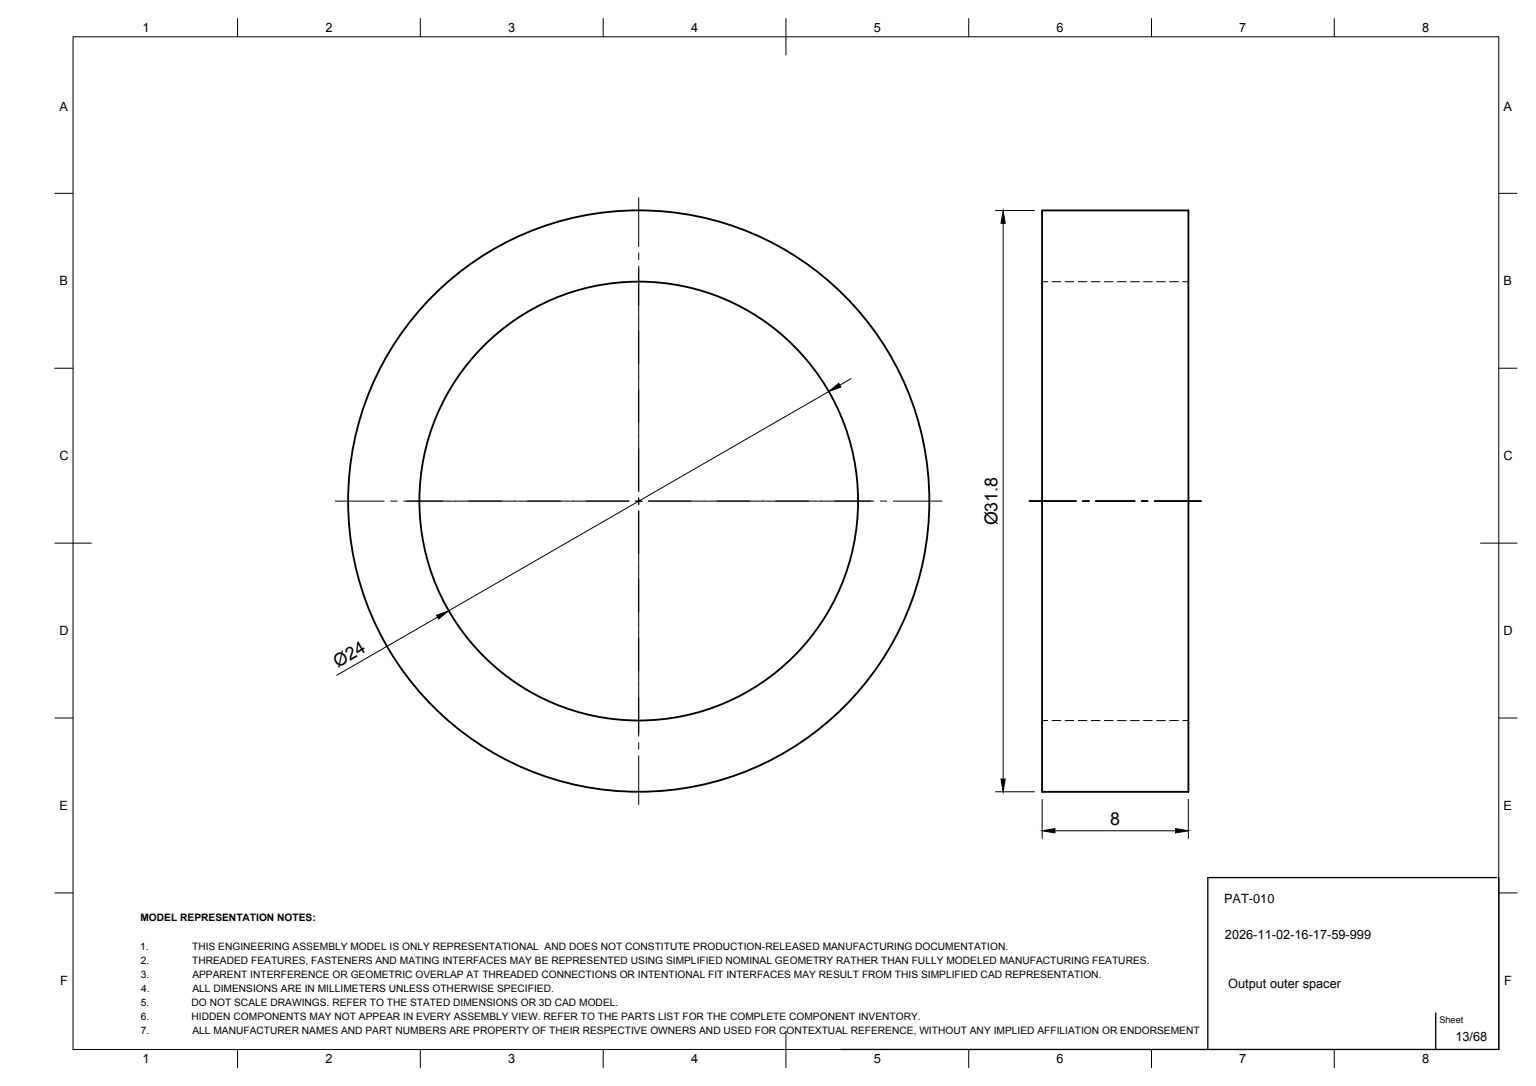
ISO-10303-21;
HEADER;
/* Generated by software containing ST-Developer
 * from STEP Tools, Inc. (www.steptools.com) 
 */

FILE_DESCRIPTION(
/* description */ ('Belt conveyor head drive unit'),
/* implementation_level */ '2;1');

FILE_NAME(
/* name */ 'Output outer spacer.step',
/* time_stamp */ '2026-10-28T03:26:19-07:00',
/* author */ (''),
/* organization */ (''),
/* preprocessor_version */ 'ST-DEVELOPER v20.2',
/* originating_system */ 'Autodesk Translation Framework v15.17.0.0',
/* authorisation */ '');

FILE_SCHEMA (('AUTOMOTIVE_DESIGN { 1 0 10303 214 3 1 1 }'));
ENDSEC;

DATA;
#10=MECHANICAL_DESIGN_GEOMETRIC_PRESENTATION_REPRESENTATION('',(#859),#27069);
#721=SHAPE_REPRESENTATION_RELATIONSHIP('SRR','None',#27365,#790);
#790=ADVANCED_BREP_SHAPE_REPRESENTATION('',(#944),#27007);
#859=STYLED_ITEM('',(#27811),#944);
#944=MANIFOLD_SOLID_BREP('Body1',#13724);
#1084=FACE_BOUND('',#2660,.T.);
#1085=FACE_BOUND('',#2662,.T.);
#1356=PLANE('',#14885);
#1357=PLANE('',#14886);
#1785=FACE_OUTER_BOUND('',#2657,.T.);
#1786=FACE_OUTER_BOUND('',#2658,.T.);
#1787=FACE_OUTER_BOUND('',#2659,.T.);
#1788=FACE_OUTER_BOUND('',#2661,.T.);
#2657=EDGE_LOOP('',(#9642,#9643,#9644,#9645));
#2658=EDGE_LOOP('',(#9646,#9647,#9648,#9649));
#2659=EDGE_LOOP('',(#9650));
#2660=EDGE_LOOP('',(#9651));
#2661=EDGE_LOOP('',(#9652));
#2662=EDGE_LOOP('',(#9653));
#3690=LINE('',#21711,#4482);
#3691=LINE('',#21717,#4483);
#4482=VECTOR('',#17264,1.2);
#4483=VECTOR('',#17271,1.59);
#5232=CIRCLE('',#14880,1.2);
#5233=CIRCLE('',#14881,1.2);
#5234=CIRCLE('',#14883,1.59);
#5235=CIRCLE('',#14884,1.59);
#6181=VERTEX_POINT('',#21708);
#6182=VERTEX_POINT('',#21710);
#6183=VERTEX_POINT('',#21714);
#6184=VERTEX_POINT('',#21716);
#7513=EDGE_CURVE('',#6181,#6181,#5232,.T.);
#7514=EDGE_CURVE('',#6181,#6182,#3690,.T.);
#7515=EDGE_CURVE('',#6182,#6182,#5233,.T.);
#7516=EDGE_CURVE('',#6183,#6183,#5234,.T.);
#7517=EDGE_CURVE('',#6183,#6184,#3691,.T.);
#7518=EDGE_CURVE('',#6184,#6184,#5235,.T.);
#9642=ORIENTED_EDGE('',*,*,#7513,.F.);
#9643=ORIENTED_EDGE('',*,*,#7514,.T.);
#9644=ORIENTED_EDGE('',*,*,#7515,.T.);
#9645=ORIENTED_EDGE('',*,*,#7514,.F.);
#9646=ORIENTED_EDGE('',*,*,#7516,.F.);
#9647=ORIENTED_EDGE('',*,*,#7517,.T.);
#9648=ORIENTED_EDGE('',*,*,#7518,.T.);
#9649=ORIENTED_EDGE('',*,*,#7517,.F.);
#9650=ORIENTED_EDGE('',*,*,#7516,.T.);
#9651=ORIENTED_EDGE('',*,*,#7513,.T.);
#9652=ORIENTED_EDGE('',*,*,#7518,.F.);
#9653=ORIENTED_EDGE('',*,*,#7515,.F.);
#12605=CYLINDRICAL_SURFACE('',#14879,1.2);
#12606=CYLINDRICAL_SURFACE('',#14882,1.59);
#13064=ADVANCED_FACE('',(#1785),#12605,.F.);
#13065=ADVANCED_FACE('',(#1786),#12606,.T.);
#13066=ADVANCED_FACE('',(#1787,#1084),#1356,.T.);
#13067=ADVANCED_FACE('',(#1788,#1085),#1357,.F.);
#13724=CLOSED_SHELL('',(#13064,#13065,#13066,#13067));
#14878=AXIS2_PLACEMENT_3D('',#21706,#17258,#17259);
#14879=AXIS2_PLACEMENT_3D('',#21707,#17260,#17261);
#14880=AXIS2_PLACEMENT_3D('',#21709,#17262,#17263);
#14881=AXIS2_PLACEMENT_3D('',#21712,#17265,#17266);
#14882=AXIS2_PLACEMENT_3D('',#21713,#17267,#17268);
#14883=AXIS2_PLACEMENT_3D('',#21715,#17269,#17270);
#14884=AXIS2_PLACEMENT_3D('',#21718,#17272,#17273);
#14885=AXIS2_PLACEMENT_3D('',#21719,#17274,#17275);
#14886=AXIS2_PLACEMENT_3D('',#21720,#17276,#17277);
#17258=DIRECTION('axis',(0.,0.,1.));
#17259=DIRECTION('refdir',(1.,0.,0.));
#17260=DIRECTION('center_axis',(0.,1.,0.));
#17261=DIRECTION('ref_axis',(1.,0.,0.));
#17262=DIRECTION('center_axis',(0.,-1.,0.));
#17263=DIRECTION('ref_axis',(1.,0.,0.));
#17264=DIRECTION('',(0.,-1.,0.));
#17265=DIRECTION('center_axis',(0.,-1.,0.));
#17266=DIRECTION('ref_axis',(1.,0.,0.));
#17267=DIRECTION('center_axis',(0.,1.,0.));
#17268=DIRECTION('ref_axis',(1.,0.,0.));
#17269=DIRECTION('center_axis',(0.,1.,0.));
#17270=DIRECTION('ref_axis',(1.,0.,0.));
#17271=DIRECTION('',(0.,-1.,0.));
#17272=DIRECTION('center_axis',(0.,1.,0.));
#17273=DIRECTION('ref_axis',(1.,0.,0.));
#17274=DIRECTION('center_axis',(0.,1.,0.));
#17275=DIRECTION('ref_axis',(1.,0.,0.));
#17276=DIRECTION('center_axis',(0.,1.,0.));
#17277=DIRECTION('ref_axis',(1.,0.,0.));
#21706=CARTESIAN_POINT('',(0.,0.,0.));
#21707=CARTESIAN_POINT('Origin',(6.97091003018116,-0.4,7.));
#21708=CARTESIAN_POINT('',(5.77091003018116,0.4,7.));
#21709=CARTESIAN_POINT('Origin',(6.97091003018116,0.4,7.));
#21710=CARTESIAN_POINT('',(5.77091003018116,-0.4,7.));
#21711=CARTESIAN_POINT('',(5.77091003018116,-0.4,7.));
#21712=CARTESIAN_POINT('Origin',(6.97091003018116,-0.4,7.));
#21713=CARTESIAN_POINT('Origin',(6.97091003018116,-0.4,7.));
#21714=CARTESIAN_POINT('',(5.38091003018116,0.4,7.));
#21715=CARTESIAN_POINT('Origin',(6.97091003018116,0.4,7.));
#21716=CARTESIAN_POINT('',(5.38091003018116,-0.4,7.));
#21717=CARTESIAN_POINT('',(5.38091003018116,-0.4,7.));
#21718=CARTESIAN_POINT('Origin',(6.97091003018116,-0.4,7.));
#21719=CARTESIAN_POINT('Origin',(6.97091003018116,0.4,7.));
#21720=CARTESIAN_POINT('Origin',(6.97091003018116,-0.4,7.));
#26930=UNCERTAINTY_MEASURE_WITH_UNIT(LENGTH_MEASURE(0.001),#27070,
'DISTANCE_ACCURACY_VALUE',
'Maximum model space distance between geometric entities at asserted c
onnectivities');
#26992=UNCERTAINTY_MEASURE_WITH_UNIT(LENGTH_MEASURE(0.001),#27070,
'DISTANCE_ACCURACY_VALUE',
'Maximum model space distance between geometric entities at asserted c
onnectivities');
#27007=(
GEOMETRIC_REPRESENTATION_CONTEXT(3)
GLOBAL_UNCERTAINTY_ASSIGNED_CONTEXT((#26930))
GLOBAL_UNIT_ASSIGNED_CONTEXT((#27070,#27072,#27073))
REPRESENTATION_CONTEXT('','3D')
);
#27069=(
GEOMETRIC_REPRESENTATION_CONTEXT(3)
GLOBAL_UNCERTAINTY_ASSIGNED_CONTEXT((#26992))
GLOBAL_UNIT_ASSIGNED_CONTEXT((#27070,#27072,#27073))
REPRESENTATION_CONTEXT('','3D')
);
#27070=(
LENGTH_UNIT()
NAMED_UNIT(*)
SI_UNIT(.CENTI.,.METRE.)
);
#27072=(
NAMED_UNIT(*)
PLANE_ANGLE_UNIT()
SI_UNIT($,.RADIAN.)
);
#27073=(
NAMED_UNIT(*)
SI_UNIT($,.STERADIAN.)
SOLID_ANGLE_UNIT()
);
#27088=SHAPE_DEFINITION_REPRESENTATION(#27164,#27365);
#27164=PRODUCT_DEFINITION_SHAPE('',$,#27442);
#27365=SHAPE_REPRESENTATION('',(#14878),#27007);
#27427=PRODUCT_DEFINITION_CONTEXT('part definition',#27657,'design');
#27442=PRODUCT_DEFINITION('Output outer spacer','Output outer spacer',#27518,
#27427);
#27518=PRODUCT_DEFINITION_FORMATION('',$,#27673);
#27657=APPLICATION_CONTEXT(
'Core Data for Automotive Mechanical Design Process');
#27658=PRODUCT_CONTEXT('part definition',#27657,'mechanical');
#27673=PRODUCT('Output outer spacer','Output outer spacer',
'Output outer spacer',(#27658));
#27805=COLOUR_RGB('Off White',0.89,0.88,0.83);
#27806=FILL_AREA_STYLE_COLOUR('',#27805);
#27807=FILL_AREA_STYLE('',(#27806));
#27808=SURFACE_STYLE_FILL_AREA(#27807);
#27809=SURFACE_SIDE_STYLE('',(#27808));
#27810=SURFACE_STYLE_USAGE(.BOTH.,#27809);
#27811=PRESENTATION_STYLE_ASSIGNMENT((#27810));
ENDSEC;
END-ISO-10303-21;
